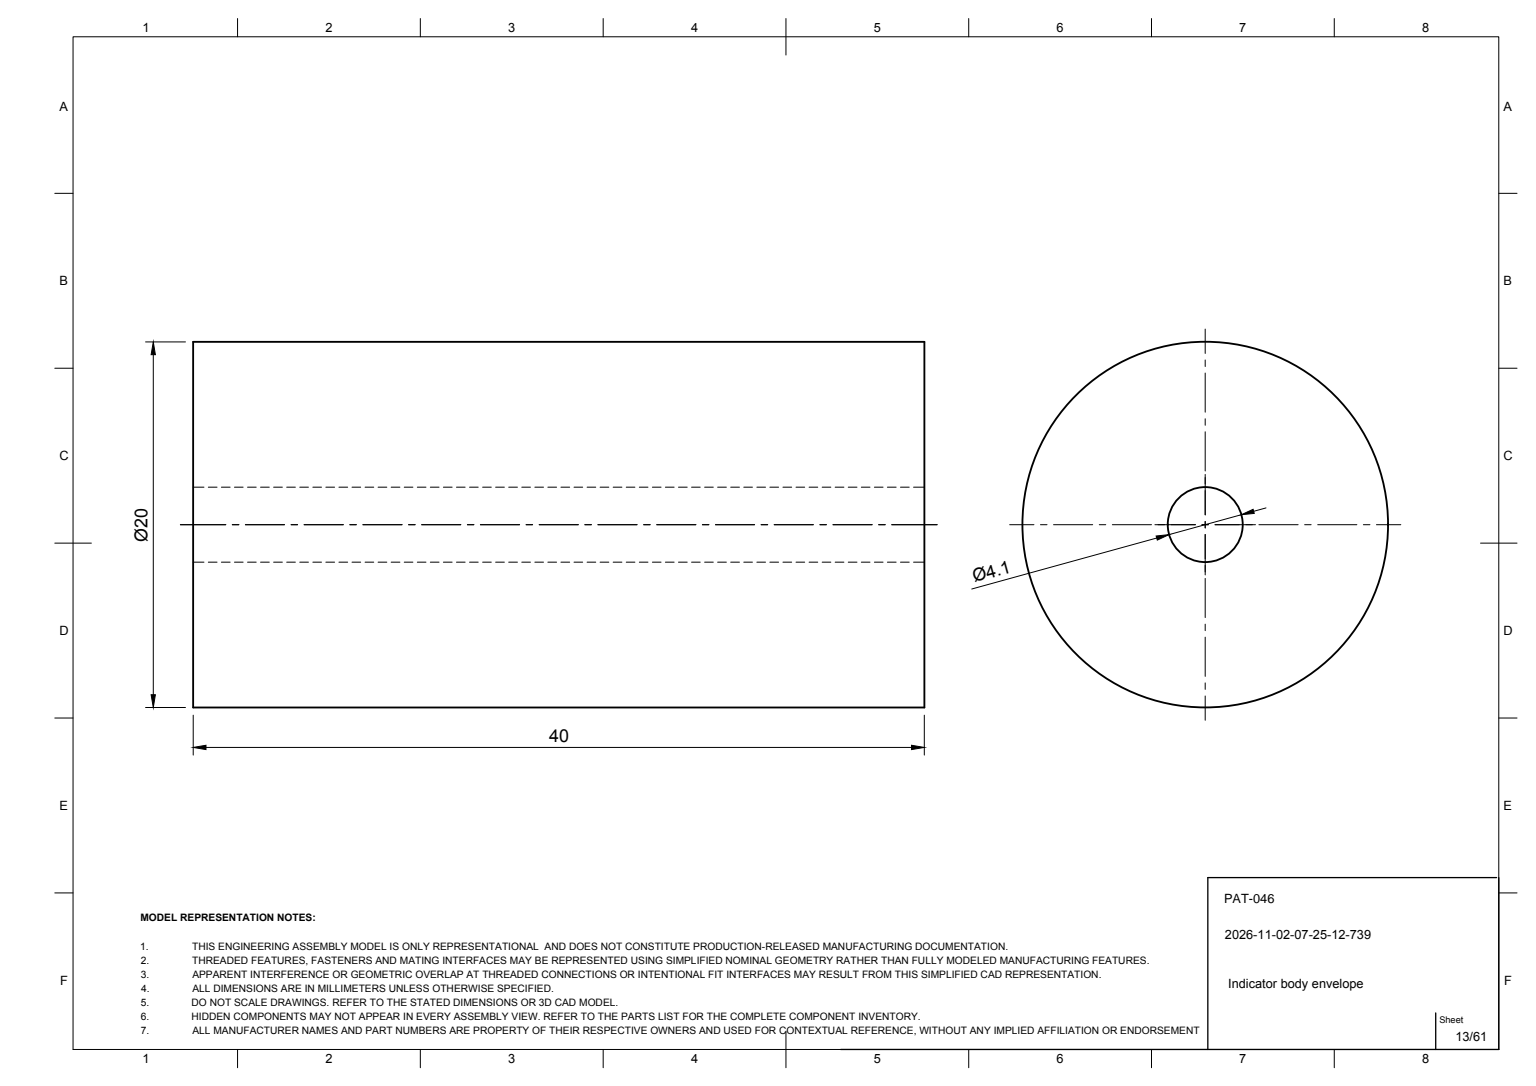
ISO-10303-21;
HEADER;
/* Generated by software containing ST-Developer
 * from STEP Tools, Inc. (www.steptools.com) 
 */

FILE_DESCRIPTION(
/* description */ ('Gear mesh backlash fixture'),
/* implementation_level */ '2;1');

FILE_NAME(
/* name */ 'Indicator body envelope.step',
/* time_stamp */ '2026-10-28T03:26:00-07:00',
/* author */ (''),
/* organization */ (''),
/* preprocessor_version */ 'ST-DEVELOPER v20.2',
/* originating_system */ 'Autodesk Translation Framework v15.17.0.0',
/* authorisation */ '');

FILE_SCHEMA (('AUTOMOTIVE_DESIGN { 1 0 10303 214 3 1 1 }'));
ENDSEC;

DATA;
#10=MECHANICAL_DESIGN_GEOMETRIC_PRESENTATION_REPRESENTATION('',(#1024),#57900);
#924=SHAPE_REPRESENTATION_RELATIONSHIP('SRR','None',#58119,#974);
#974=ADVANCED_BREP_SHAPE_REPRESENTATION('',(#1089),#57852);
#1024=STYLED_ITEM('',(#58444),#1089);
#1089=MANIFOLD_SOLID_BREP('Body1',#13584);
#1203=FACE_BOUND('',#2632,.T.);
#1204=FACE_BOUND('',#2634,.T.);
#1389=PLANE('',#14439);
#1390=PLANE('',#14440);
#1804=FACE_OUTER_BOUND('',#2629,.T.);
#1805=FACE_OUTER_BOUND('',#2630,.T.);
#1806=FACE_OUTER_BOUND('',#2631,.T.);
#1807=FACE_OUTER_BOUND('',#2633,.T.);
#2629=EDGE_LOOP('',(#9403,#9404,#9405,#9406));
#2630=EDGE_LOOP('',(#9407,#9408,#9409,#9410));
#2631=EDGE_LOOP('',(#9411));
#2632=EDGE_LOOP('',(#9412));
#2633=EDGE_LOOP('',(#9413));
#2634=EDGE_LOOP('',(#9414));
#3549=LINE('',#19885,#4438);
#3550=LINE('',#19891,#4439);
#4438=VECTOR('',#16196,0.205);
#4439=VECTOR('',#16203,1.);
#5306=CIRCLE('',#14434,0.205);
#5307=CIRCLE('',#14435,0.205);
#5308=CIRCLE('',#14437,1.);
#5309=CIRCLE('',#14438,1.);
#5951=VERTEX_POINT('',#19882);
#5952=VERTEX_POINT('',#19884);
#5953=VERTEX_POINT('',#19888);
#5954=VERTEX_POINT('',#19890);
#7288=EDGE_CURVE('',#5951,#5951,#5306,.T.);
#7289=EDGE_CURVE('',#5951,#5952,#3549,.T.);
#7290=EDGE_CURVE('',#5952,#5952,#5307,.T.);
#7291=EDGE_CURVE('',#5953,#5953,#5308,.T.);
#7292=EDGE_CURVE('',#5953,#5954,#3550,.T.);
#7293=EDGE_CURVE('',#5954,#5954,#5309,.T.);
#9403=ORIENTED_EDGE('',*,*,#7288,.F.);
#9404=ORIENTED_EDGE('',*,*,#7289,.T.);
#9405=ORIENTED_EDGE('',*,*,#7290,.T.);
#9406=ORIENTED_EDGE('',*,*,#7289,.F.);
#9407=ORIENTED_EDGE('',*,*,#7291,.F.);
#9408=ORIENTED_EDGE('',*,*,#7292,.T.);
#9409=ORIENTED_EDGE('',*,*,#7293,.T.);
#9410=ORIENTED_EDGE('',*,*,#7292,.F.);
#9411=ORIENTED_EDGE('',*,*,#7291,.T.);
#9412=ORIENTED_EDGE('',*,*,#7288,.T.);
#9413=ORIENTED_EDGE('',*,*,#7293,.F.);
#9414=ORIENTED_EDGE('',*,*,#7290,.F.);
#12636=CYLINDRICAL_SURFACE('',#14433,0.205);
#12637=CYLINDRICAL_SURFACE('',#14436,1.);
#12921=ADVANCED_FACE('',(#1804),#12636,.F.);
#12922=ADVANCED_FACE('',(#1805),#12637,.T.);
#12923=ADVANCED_FACE('',(#1806,#1203),#1389,.T.);
#12924=ADVANCED_FACE('',(#1807,#1204),#1390,.F.);
#13584=CLOSED_SHELL('',(#12921,#12922,#12923,#12924));
#14432=AXIS2_PLACEMENT_3D('',#19880,#16190,#16191);
#14433=AXIS2_PLACEMENT_3D('',#19881,#16192,#16193);
#14434=AXIS2_PLACEMENT_3D('',#19883,#16194,#16195);
#14435=AXIS2_PLACEMENT_3D('',#19886,#16197,#16198);
#14436=AXIS2_PLACEMENT_3D('',#19887,#16199,#16200);
#14437=AXIS2_PLACEMENT_3D('',#19889,#16201,#16202);
#14438=AXIS2_PLACEMENT_3D('',#19892,#16204,#16205);
#14439=AXIS2_PLACEMENT_3D('',#19893,#16206,#16207);
#14440=AXIS2_PLACEMENT_3D('',#19894,#16208,#16209);
#16190=DIRECTION('axis',(0.,0.,1.));
#16191=DIRECTION('refdir',(1.,0.,0.));
#16192=DIRECTION('center_axis',(0.,1.,0.));
#16193=DIRECTION('ref_axis',(1.,0.,0.));
#16194=DIRECTION('center_axis',(0.,-1.,0.));
#16195=DIRECTION('ref_axis',(1.,0.,0.));
#16196=DIRECTION('',(0.,-1.,0.));
#16197=DIRECTION('center_axis',(0.,-1.,0.));
#16198=DIRECTION('ref_axis',(1.,0.,0.));
#16199=DIRECTION('center_axis',(0.,1.,0.));
#16200=DIRECTION('ref_axis',(1.,0.,0.));
#16201=DIRECTION('center_axis',(0.,1.,0.));
#16202=DIRECTION('ref_axis',(1.,0.,0.));
#16203=DIRECTION('',(0.,-1.,0.));
#16204=DIRECTION('center_axis',(0.,1.,0.));
#16205=DIRECTION('ref_axis',(1.,0.,0.));
#16206=DIRECTION('center_axis',(0.,1.,0.));
#16207=DIRECTION('ref_axis',(1.,0.,0.));
#16208=DIRECTION('center_axis',(0.,1.,0.));
#16209=DIRECTION('ref_axis',(1.,0.,0.));
#19880=CARTESIAN_POINT('',(0.,0.,0.));
#19881=CARTESIAN_POINT('Origin',(6.,6.,12.));
#19882=CARTESIAN_POINT('',(5.795,10.,12.));
#19883=CARTESIAN_POINT('Origin',(6.,10.,12.));
#19884=CARTESIAN_POINT('',(5.795,6.,12.));
#19885=CARTESIAN_POINT('',(5.795,6.,12.));
#19886=CARTESIAN_POINT('Origin',(6.,6.,12.));
#19887=CARTESIAN_POINT('Origin',(6.,6.,12.));
#19888=CARTESIAN_POINT('',(5.,10.,12.));
#19889=CARTESIAN_POINT('Origin',(6.,10.,12.));
#19890=CARTESIAN_POINT('',(5.,6.,12.));
#19891=CARTESIAN_POINT('',(5.,6.,12.));
#19892=CARTESIAN_POINT('Origin',(6.,6.,12.));
#19893=CARTESIAN_POINT('Origin',(6.,10.,12.));
#19894=CARTESIAN_POINT('Origin',(6.,6.,12.));
#57793=UNCERTAINTY_MEASURE_WITH_UNIT(LENGTH_MEASURE(0.001),#57901,
'DISTANCE_ACCURACY_VALUE',
'Maximum model space distance between geometric entities at asserted c
onnectivities');
#57841=UNCERTAINTY_MEASURE_WITH_UNIT(LENGTH_MEASURE(0.001),#57901,
'DISTANCE_ACCURACY_VALUE',
'Maximum model space distance between geometric entities at asserted c
onnectivities');
#57852=(
GEOMETRIC_REPRESENTATION_CONTEXT(3)
GLOBAL_UNCERTAINTY_ASSIGNED_CONTEXT((#57793))
GLOBAL_UNIT_ASSIGNED_CONTEXT((#57901,#57903,#57904))
REPRESENTATION_CONTEXT('','3D')
);
#57900=(
GEOMETRIC_REPRESENTATION_CONTEXT(3)
GLOBAL_UNCERTAINTY_ASSIGNED_CONTEXT((#57841))
GLOBAL_UNIT_ASSIGNED_CONTEXT((#57901,#57903,#57904))
REPRESENTATION_CONTEXT('','3D')
);
#57901=(
LENGTH_UNIT()
NAMED_UNIT(*)
SI_UNIT(.CENTI.,.METRE.)
);
#57903=(
NAMED_UNIT(*)
PLANE_ANGLE_UNIT()
SI_UNIT($,.RADIAN.)
);
#57904=(
NAMED_UNIT(*)
SI_UNIT($,.STERADIAN.)
SOLID_ANGLE_UNIT()
);
#57915=SHAPE_DEFINITION_REPRESENTATION(#57973,#58119);
#57973=PRODUCT_DEFINITION_SHAPE('',$,#58178);
#58119=SHAPE_REPRESENTATION('',(#14432),#57852);
#58167=PRODUCT_DEFINITION_CONTEXT('part definition',#58343,'design');
#58178=PRODUCT_DEFINITION('Indicator body envelope',
'Indicator body envelope',#58236,#58167);
#58236=PRODUCT_DEFINITION_FORMATION('',$,#58355);
#58343=APPLICATION_CONTEXT(
'Core Data for Automotive Mechanical Design Process');
#58344=PRODUCT_CONTEXT('part definition',#58343,'mechanical');
#58355=PRODUCT('Indicator body envelope','Indicator body envelope',
'Indicator body envelope',(#58344));
#58438=COLOUR_RGB('Dark Blue',0.08,0.2,0.34);
#58439=FILL_AREA_STYLE_COLOUR('',#58438);
#58440=FILL_AREA_STYLE('',(#58439));
#58441=SURFACE_STYLE_FILL_AREA(#58440);
#58442=SURFACE_SIDE_STYLE('',(#58441));
#58443=SURFACE_STYLE_USAGE(.BOTH.,#58442);
#58444=PRESENTATION_STYLE_ASSIGNMENT((#58443));
ENDSEC;
END-ISO-10303-21;
